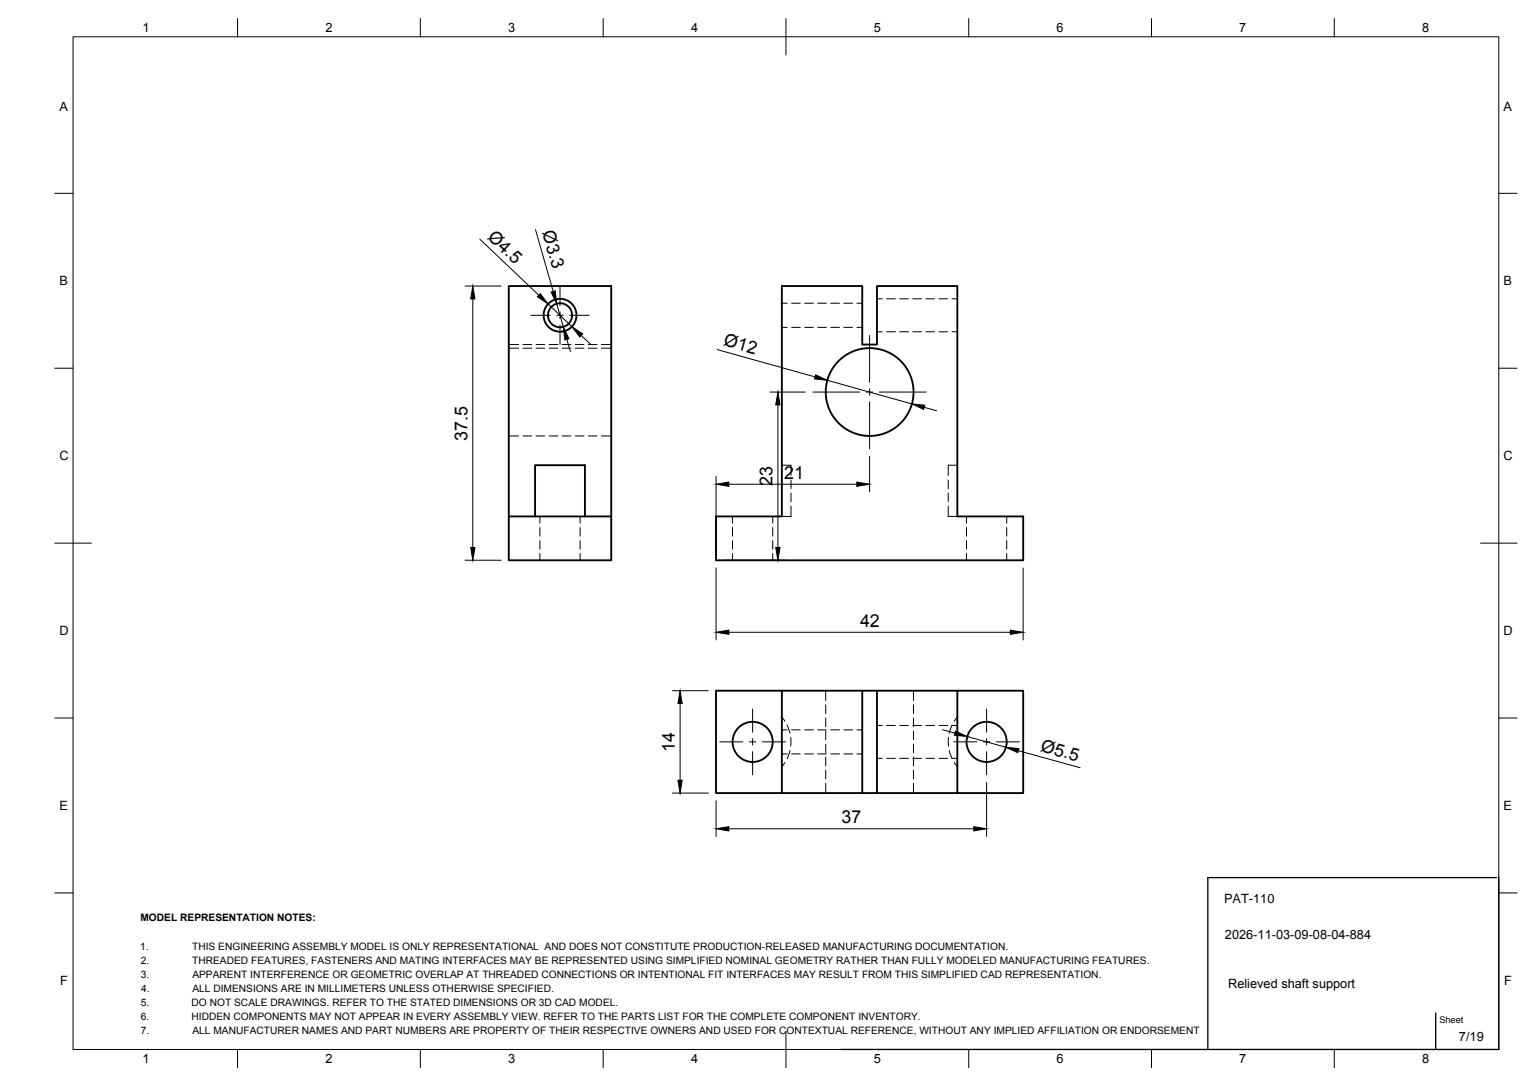
ISO-10303-21;
HEADER;
/* Generated by software containing ST-Developer
 * from STEP Tools, Inc. (www.steptools.com) 
 */

FILE_DESCRIPTION(
/* description */ ('Twin-shaft manual slide'),
/* implementation_level */ '2;1');

FILE_NAME(
/* name */ 'Relieved shaft support.step',
/* time_stamp */ '2026-10-27T18:38:08-07:00',
/* author */ (''),
/* organization */ (''),
/* preprocessor_version */ 'ST-DEVELOPER v20.2',
/* originating_system */ 'Autodesk Translation Framework v15.17.0.0',
/* authorisation */ '');

FILE_SCHEMA (('AUTOMOTIVE_DESIGN { 1 0 10303 214 3 1 1 }'));
ENDSEC;

DATA;
#10=MECHANICAL_DESIGN_GEOMETRIC_PRESENTATION_REPRESENTATION('',(#278),#6463);
#246=SHAPE_REPRESENTATION_RELATIONSHIP('SRR','None',#6564,#262);
#262=ADVANCED_BREP_SHAPE_REPRESENTATION('',(#294),#6447);
#278=STYLED_ITEM('',(#6740),#294);
#294=MANIFOLD_SOLID_BREP('Body1',#3640);
#328=FACE_BOUND('',#785,.T.);
#329=FACE_BOUND('',#787,.T.);
#330=FACE_BOUND('',#789,.T.);
#331=FACE_BOUND('',#796,.T.);
#332=FACE_BOUND('',#799,.T.);
#333=FACE_BOUND('',#800,.T.);
#334=FACE_BOUND('',#803,.T.);
#335=FACE_BOUND('',#806,.T.);
#336=FACE_BOUND('',#809,.T.);
#337=FACE_BOUND('',#812,.T.);
#409=PLANE('',#3891);
#410=PLANE('',#3898);
#411=PLANE('',#3899);
#412=PLANE('',#3901);
#413=PLANE('',#3903);
#414=PLANE('',#3917);
#415=PLANE('',#3918);
#416=PLANE('',#3919);
#417=PLANE('',#3920);
#418=PLANE('',#3921);
#419=PLANE('',#3922);
#420=PLANE('',#3923);
#421=PLANE('',#3924);
#422=PLANE('',#3925);
#423=PLANE('',#3926);
#424=PLANE('',#3927);
#549=FACE_OUTER_BOUND('',#780,.T.);
#550=FACE_OUTER_BOUND('',#781,.T.);
#551=FACE_OUTER_BOUND('',#782,.T.);
#552=FACE_OUTER_BOUND('',#783,.T.);
#553=FACE_OUTER_BOUND('',#784,.T.);
#554=FACE_OUTER_BOUND('',#786,.T.);
#555=FACE_OUTER_BOUND('',#788,.T.);
#556=FACE_OUTER_BOUND('',#790,.T.);
#557=FACE_OUTER_BOUND('',#791,.T.);
#558=FACE_OUTER_BOUND('',#792,.T.);
#559=FACE_OUTER_BOUND('',#793,.T.);
#560=FACE_OUTER_BOUND('',#794,.T.);
#561=FACE_OUTER_BOUND('',#795,.T.);
#562=FACE_OUTER_BOUND('',#797,.T.);
#563=FACE_OUTER_BOUND('',#798,.T.);
#564=FACE_OUTER_BOUND('',#801,.T.);
#565=FACE_OUTER_BOUND('',#802,.T.);
#566=FACE_OUTER_BOUND('',#804,.T.);
#567=FACE_OUTER_BOUND('',#805,.T.);
#568=FACE_OUTER_BOUND('',#807,.T.);
#569=FACE_OUTER_BOUND('',#808,.T.);
#570=FACE_OUTER_BOUND('',#810,.T.);
#571=FACE_OUTER_BOUND('',#811,.T.);
#780=EDGE_LOOP('',(#2598,#2599));
#781=EDGE_LOOP('',(#2600,#2601,#2602,#2603));
#782=EDGE_LOOP('',(#2604,#2605,#2606,#2607));
#783=EDGE_LOOP('',(#2608,#2609));
#784=EDGE_LOOP('',(#2610,#2611,#2612,#2613,#2614,#2615));
#785=EDGE_LOOP('',(#2616));
#786=EDGE_LOOP('',(#2617,#2618,#2619,#2620,#2621,#2622,#2623,#2624));
#787=EDGE_LOOP('',(#2625));
#788=EDGE_LOOP('',(#2626,#2627,#2628,#2629,#2630,#2631));
#789=EDGE_LOOP('',(#2632));
#790=EDGE_LOOP('',(#2633,#2634,#2635,#2636));
#791=EDGE_LOOP('',(#2637,#2638,#2639,#2640));
#792=EDGE_LOOP('',(#2641,#2642,#2643,#2644));
#793=EDGE_LOOP('',(#2645,#2646,#2647,#2648));
#794=EDGE_LOOP('',(#2649,#2650,#2651,#2652));
#795=EDGE_LOOP('',(#2653,#2654,#2655,#2656,#2657,#2658,#2659,#2660,#2661,
#2662,#2663,#2664));
#796=EDGE_LOOP('',(#2665));
#797=EDGE_LOOP('',(#2666,#2667,#2668,#2669));
#798=EDGE_LOOP('',(#2670,#2671,#2672,#2673));
#799=EDGE_LOOP('',(#2674));
#800=EDGE_LOOP('',(#2675));
#801=EDGE_LOOP('',(#2676,#2677,#2678,#2679));
#802=EDGE_LOOP('',(#2680,#2681,#2682,#2683,#2684,#2685,#2686,#2687));
#803=EDGE_LOOP('',(#2688));
#804=EDGE_LOOP('',(#2689,#2690,#2691,#2692));
#805=EDGE_LOOP('',(#2693,#2694,#2695,#2696));
#806=EDGE_LOOP('',(#2697));
#807=EDGE_LOOP('',(#2698,#2699,#2700,#2701));
#808=EDGE_LOOP('',(#2702,#2703,#2704,#2705));
#809=EDGE_LOOP('',(#2706));
#810=EDGE_LOOP('',(#2707,#2708,#2709,#2710));
#811=EDGE_LOOP('',(#2711,#2712,#2713,#2714,#2715,#2716,#2717,#2718,#2719,
#2720,#2721,#2722));
#812=EDGE_LOOP('',(#2723));
#1064=LINE('',#5539,#1350);
#1065=LINE('',#5543,#1351);
#1066=LINE('',#5546,#1352);
#1067=LINE('',#5550,#1353);
#1068=LINE('',#5554,#1354);
#1069=LINE('',#5557,#1355);
#1070=LINE('',#5560,#1356);
#1071=LINE('',#5562,#1357);
#1072=LINE('',#5564,#1358);
#1073=LINE('',#5566,#1359);
#1074=LINE('',#5567,#1360);
#1075=LINE('',#5572,#1361);
#1076=LINE('',#5574,#1362);
#1077=LINE('',#5575,#1363);
#1078=LINE('',#5581,#1364);
#1079=LINE('',#5583,#1365);
#1080=LINE('',#5584,#1366);
#1081=LINE('',#5586,#1367);
#1082=LINE('',#5587,#1368);
#1083=LINE('',#5594,#1369);
#1084=LINE('',#5598,#1370);
#1085=LINE('',#5603,#1371);
#1086=LINE('',#5607,#1372);
#1087=LINE('',#5612,#1373);
#1088=LINE('',#5616,#1374);
#1089=LINE('',#5618,#1375);
#1090=LINE('',#5619,#1376);
#1091=LINE('',#5621,#1377);
#1092=LINE('',#5623,#1378);
#1093=LINE('',#5625,#1379);
#1094=LINE('',#5627,#1380);
#1095=LINE('',#5629,#1381);
#1096=LINE('',#5630,#1382);
#1097=LINE('',#5633,#1383);
#1098=LINE('',#5634,#1384);
#1099=LINE('',#5637,#1385);
#1100=LINE('',#5638,#1386);
#1101=LINE('',#5640,#1387);
#1102=LINE('',#5643,#1388);
#1103=LINE('',#5644,#1389);
#1104=LINE('',#5647,#1390);
#1105=LINE('',#5648,#1391);
#1106=LINE('',#5651,#1392);
#1107=LINE('',#5652,#1393);
#1108=LINE('',#5655,#1394);
#1109=LINE('',#5656,#1395);
#1110=LINE('',#5659,#1396);
#1111=LINE('',#5660,#1397);
#1112=LINE('',#5662,#1398);
#1350=VECTOR('',#4408,1.);
#1351=VECTOR('',#4413,1.);
#1352=VECTOR('',#4416,1.);
#1353=VECTOR('',#4419,1.);
#1354=VECTOR('',#4422,1.);
#1355=VECTOR('',#4427,1.);
#1356=VECTOR('',#4430,1.);
#1357=VECTOR('',#4431,1.);
#1358=VECTOR('',#4432,1.);
#1359=VECTOR('',#4433,1.);
#1360=VECTOR('',#4434,1.);
#1361=VECTOR('',#4439,1.);
#1362=VECTOR('',#4440,1.);
#1363=VECTOR('',#4441,1.);
#1364=VECTOR('',#4446,1.);
#1365=VECTOR('',#4447,1.);
#1366=VECTOR('',#4448,1.);
#1367=VECTOR('',#4449,1.);
#1368=VECTOR('',#4450,1.);
#1369=VECTOR('',#4457,0.225);
#1370=VECTOR('',#4462,0.165);
#1371=VECTOR('',#4469,0.275);
#1372=VECTOR('',#4474,0.275);
#1373=VECTOR('',#4479,0.6);
#1374=VECTOR('',#4484,1.);
#1375=VECTOR('',#4485,1.);
#1376=VECTOR('',#4486,1.);
#1377=VECTOR('',#4487,1.);
#1378=VECTOR('',#4488,1.);
#1379=VECTOR('',#4489,1.);
#1380=VECTOR('',#4490,1.);
#1381=VECTOR('',#4491,1.);
#1382=VECTOR('',#4492,1.);
#1383=VECTOR('',#4495,1.);
#1384=VECTOR('',#4496,1.);
#1385=VECTOR('',#4499,1.);
#1386=VECTOR('',#4500,1.);
#1387=VECTOR('',#4503,1.);
#1388=VECTOR('',#4506,1.);
#1389=VECTOR('',#4507,1.);
#1390=VECTOR('',#4510,1.);
#1391=VECTOR('',#4511,1.);
#1392=VECTOR('',#4514,1.);
#1393=VECTOR('',#4515,1.);
#1394=VECTOR('',#4518,1.);
#1395=VECTOR('',#4519,1.);
#1396=VECTOR('',#4522,1.);
#1397=VECTOR('',#4523,1.);
#1398=VECTOR('',#4526,1.);
#1637=CIRCLE('',#3892,0.525);
#1638=CIRCLE('',#3894,0.525);
#1639=CIRCLE('',#3896,0.525);
#1640=CIRCLE('',#3897,0.525);
#1641=CIRCLE('',#3900,0.275);
#1642=CIRCLE('',#3902,0.165);
#1643=CIRCLE('',#3904,0.275);
#1644=CIRCLE('',#3906,0.225);
#1645=CIRCLE('',#3907,0.225);
#1646=CIRCLE('',#3909,0.165);
#1647=CIRCLE('',#3911,0.275);
#1648=CIRCLE('',#3913,0.275);
#1649=CIRCLE('',#3915,0.6);
#1650=CIRCLE('',#3916,0.6);
#1798=VERTEX_POINT('',#5537);
#1799=VERTEX_POINT('',#5538);
#1800=VERTEX_POINT('',#5542);
#1801=VERTEX_POINT('',#5544);
#1802=VERTEX_POINT('',#5548);
#1803=VERTEX_POINT('',#5549);
#1804=VERTEX_POINT('',#5551);
#1805=VERTEX_POINT('',#5553);
#1806=VERTEX_POINT('',#5559);
#1807=VERTEX_POINT('',#5561);
#1808=VERTEX_POINT('',#5563);
#1809=VERTEX_POINT('',#5565);
#1810=VERTEX_POINT('',#5568);
#1811=VERTEX_POINT('',#5571);
#1812=VERTEX_POINT('',#5573);
#1813=VERTEX_POINT('',#5576);
#1814=VERTEX_POINT('',#5579);
#1815=VERTEX_POINT('',#5580);
#1816=VERTEX_POINT('',#5582);
#1817=VERTEX_POINT('',#5585);
#1818=VERTEX_POINT('',#5588);
#1819=VERTEX_POINT('',#5591);
#1820=VERTEX_POINT('',#5593);
#1821=VERTEX_POINT('',#5597);
#1822=VERTEX_POINT('',#5601);
#1823=VERTEX_POINT('',#5605);
#1824=VERTEX_POINT('',#5609);
#1825=VERTEX_POINT('',#5611);
#1826=VERTEX_POINT('',#5615);
#1827=VERTEX_POINT('',#5617);
#1828=VERTEX_POINT('',#5620);
#1829=VERTEX_POINT('',#5622);
#1830=VERTEX_POINT('',#5624);
#1831=VERTEX_POINT('',#5626);
#1832=VERTEX_POINT('',#5628);
#1833=VERTEX_POINT('',#5632);
#1834=VERTEX_POINT('',#5636);
#1835=VERTEX_POINT('',#5642);
#1836=VERTEX_POINT('',#5646);
#1837=VERTEX_POINT('',#5650);
#1838=VERTEX_POINT('',#5654);
#1839=VERTEX_POINT('',#5658);
#2104=EDGE_CURVE('',#1798,#1799,#1064,.T.);
#2105=EDGE_CURVE('',#1799,#1798,#1637,.T.);
#2106=EDGE_CURVE('',#1800,#1798,#1065,.T.);
#2107=EDGE_CURVE('',#1801,#1800,#1638,.T.);
#2108=EDGE_CURVE('',#1799,#1801,#1066,.T.);
#2109=EDGE_CURVE('',#1802,#1803,#1067,.T.);
#2110=EDGE_CURVE('',#1802,#1804,#1639,.T.);
#2111=EDGE_CURVE('',#1805,#1804,#1068,.T.);
#2112=EDGE_CURVE('',#1803,#1805,#1640,.T.);
#2113=EDGE_CURVE('',#1804,#1802,#1069,.T.);
#2114=EDGE_CURVE('',#1800,#1806,#1070,.T.);
#2115=EDGE_CURVE('',#1807,#1806,#1071,.T.);
#2116=EDGE_CURVE('',#1807,#1808,#1072,.T.);
#2117=EDGE_CURVE('',#1809,#1808,#1073,.T.);
#2118=EDGE_CURVE('',#1809,#1801,#1074,.T.);
#2119=EDGE_CURVE('',#1810,#1810,#1641,.T.);
#2120=EDGE_CURVE('',#1811,#1809,#1075,.T.);
#2121=EDGE_CURVE('',#1811,#1812,#1076,.T.);
#2122=EDGE_CURVE('',#1806,#1812,#1077,.T.);
#2123=EDGE_CURVE('',#1813,#1813,#1642,.T.);
#2124=EDGE_CURVE('',#1814,#1815,#1078,.T.);
#2125=EDGE_CURVE('',#1816,#1815,#1079,.T.);
#2126=EDGE_CURVE('',#1803,#1816,#1080,.T.);
#2127=EDGE_CURVE('',#1817,#1805,#1081,.T.);
#2128=EDGE_CURVE('',#1814,#1817,#1082,.T.);
#2129=EDGE_CURVE('',#1818,#1818,#1643,.T.);
#2130=EDGE_CURVE('',#1819,#1819,#1644,.T.);
#2131=EDGE_CURVE('',#1819,#1820,#1083,.T.);
#2132=EDGE_CURVE('',#1820,#1820,#1645,.T.);
#2133=EDGE_CURVE('',#1813,#1821,#1084,.T.);
#2134=EDGE_CURVE('',#1821,#1821,#1646,.T.);
#2135=EDGE_CURVE('',#1822,#1822,#1647,.T.);
#2136=EDGE_CURVE('',#1822,#1810,#1085,.T.);
#2137=EDGE_CURVE('',#1823,#1823,#1648,.T.);
#2138=EDGE_CURVE('',#1823,#1818,#1086,.T.);
#2139=EDGE_CURVE('',#1824,#1824,#1649,.T.);
#2140=EDGE_CURVE('',#1824,#1825,#1087,.T.);
#2141=EDGE_CURVE('',#1825,#1825,#1650,.T.);
#2142=EDGE_CURVE('',#1808,#1826,#1088,.T.);
#2143=EDGE_CURVE('',#1826,#1827,#1089,.T.);
#2144=EDGE_CURVE('',#1827,#1814,#1090,.T.);
#2145=EDGE_CURVE('',#1817,#1828,#1091,.T.);
#2146=EDGE_CURVE('',#1828,#1829,#1092,.T.);
#2147=EDGE_CURVE('',#1829,#1830,#1093,.T.);
#2148=EDGE_CURVE('',#1830,#1831,#1094,.T.);
#2149=EDGE_CURVE('',#1831,#1832,#1095,.T.);
#2150=EDGE_CURVE('',#1832,#1811,#1096,.T.);
#2151=EDGE_CURVE('',#1833,#1807,#1097,.T.);
#2152=EDGE_CURVE('',#1826,#1833,#1098,.T.);
#2153=EDGE_CURVE('',#1834,#1833,#1099,.T.);
#2154=EDGE_CURVE('',#1827,#1834,#1100,.T.);
#2155=EDGE_CURVE('',#1815,#1834,#1101,.T.);
#2156=EDGE_CURVE('',#1835,#1816,#1102,.T.);
#2157=EDGE_CURVE('',#1828,#1835,#1103,.T.);
#2158=EDGE_CURVE('',#1836,#1835,#1104,.T.);
#2159=EDGE_CURVE('',#1829,#1836,#1105,.T.);
#2160=EDGE_CURVE('',#1837,#1836,#1106,.T.);
#2161=EDGE_CURVE('',#1830,#1837,#1107,.T.);
#2162=EDGE_CURVE('',#1838,#1837,#1108,.T.);
#2163=EDGE_CURVE('',#1831,#1838,#1109,.T.);
#2164=EDGE_CURVE('',#1839,#1838,#1110,.T.);
#2165=EDGE_CURVE('',#1832,#1839,#1111,.T.);
#2166=EDGE_CURVE('',#1812,#1839,#1112,.T.);
#2598=ORIENTED_EDGE('',*,*,#2104,.F.);
#2599=ORIENTED_EDGE('',*,*,#2105,.F.);
#2600=ORIENTED_EDGE('',*,*,#2106,.F.);
#2601=ORIENTED_EDGE('',*,*,#2107,.F.);
#2602=ORIENTED_EDGE('',*,*,#2108,.F.);
#2603=ORIENTED_EDGE('',*,*,#2105,.T.);
#2604=ORIENTED_EDGE('',*,*,#2109,.F.);
#2605=ORIENTED_EDGE('',*,*,#2110,.T.);
#2606=ORIENTED_EDGE('',*,*,#2111,.F.);
#2607=ORIENTED_EDGE('',*,*,#2112,.F.);
#2608=ORIENTED_EDGE('',*,*,#2113,.F.);
#2609=ORIENTED_EDGE('',*,*,#2110,.F.);
#2610=ORIENTED_EDGE('',*,*,#2114,.T.);
#2611=ORIENTED_EDGE('',*,*,#2115,.F.);
#2612=ORIENTED_EDGE('',*,*,#2116,.T.);
#2613=ORIENTED_EDGE('',*,*,#2117,.F.);
#2614=ORIENTED_EDGE('',*,*,#2118,.T.);
#2615=ORIENTED_EDGE('',*,*,#2107,.T.);
#2616=ORIENTED_EDGE('',*,*,#2119,.T.);
#2617=ORIENTED_EDGE('',*,*,#2106,.T.);
#2618=ORIENTED_EDGE('',*,*,#2104,.T.);
#2619=ORIENTED_EDGE('',*,*,#2108,.T.);
#2620=ORIENTED_EDGE('',*,*,#2118,.F.);
#2621=ORIENTED_EDGE('',*,*,#2120,.F.);
#2622=ORIENTED_EDGE('',*,*,#2121,.T.);
#2623=ORIENTED_EDGE('',*,*,#2122,.F.);
#2624=ORIENTED_EDGE('',*,*,#2114,.F.);
#2625=ORIENTED_EDGE('',*,*,#2123,.T.);
#2626=ORIENTED_EDGE('',*,*,#2124,.T.);
#2627=ORIENTED_EDGE('',*,*,#2125,.F.);
#2628=ORIENTED_EDGE('',*,*,#2126,.F.);
#2629=ORIENTED_EDGE('',*,*,#2112,.T.);
#2630=ORIENTED_EDGE('',*,*,#2127,.F.);
#2631=ORIENTED_EDGE('',*,*,#2128,.F.);
#2632=ORIENTED_EDGE('',*,*,#2129,.T.);
#2633=ORIENTED_EDGE('',*,*,#2130,.F.);
#2634=ORIENTED_EDGE('',*,*,#2131,.T.);
#2635=ORIENTED_EDGE('',*,*,#2132,.F.);
#2636=ORIENTED_EDGE('',*,*,#2131,.F.);
#2637=ORIENTED_EDGE('',*,*,#2123,.F.);
#2638=ORIENTED_EDGE('',*,*,#2133,.T.);
#2639=ORIENTED_EDGE('',*,*,#2134,.F.);
#2640=ORIENTED_EDGE('',*,*,#2133,.F.);
#2641=ORIENTED_EDGE('',*,*,#2135,.F.);
#2642=ORIENTED_EDGE('',*,*,#2136,.T.);
#2643=ORIENTED_EDGE('',*,*,#2119,.F.);
#2644=ORIENTED_EDGE('',*,*,#2136,.F.);
#2645=ORIENTED_EDGE('',*,*,#2137,.F.);
#2646=ORIENTED_EDGE('',*,*,#2138,.T.);
#2647=ORIENTED_EDGE('',*,*,#2129,.F.);
#2648=ORIENTED_EDGE('',*,*,#2138,.F.);
#2649=ORIENTED_EDGE('',*,*,#2139,.F.);
#2650=ORIENTED_EDGE('',*,*,#2140,.T.);
#2651=ORIENTED_EDGE('',*,*,#2141,.F.);
#2652=ORIENTED_EDGE('',*,*,#2140,.F.);
#2653=ORIENTED_EDGE('',*,*,#2117,.T.);
#2654=ORIENTED_EDGE('',*,*,#2142,.T.);
#2655=ORIENTED_EDGE('',*,*,#2143,.T.);
#2656=ORIENTED_EDGE('',*,*,#2144,.T.);
#2657=ORIENTED_EDGE('',*,*,#2128,.T.);
#2658=ORIENTED_EDGE('',*,*,#2145,.T.);
#2659=ORIENTED_EDGE('',*,*,#2146,.T.);
#2660=ORIENTED_EDGE('',*,*,#2147,.T.);
#2661=ORIENTED_EDGE('',*,*,#2148,.T.);
#2662=ORIENTED_EDGE('',*,*,#2149,.T.);
#2663=ORIENTED_EDGE('',*,*,#2150,.T.);
#2664=ORIENTED_EDGE('',*,*,#2120,.T.);
#2665=ORIENTED_EDGE('',*,*,#2139,.T.);
#2666=ORIENTED_EDGE('',*,*,#2116,.F.);
#2667=ORIENTED_EDGE('',*,*,#2151,.F.);
#2668=ORIENTED_EDGE('',*,*,#2152,.F.);
#2669=ORIENTED_EDGE('',*,*,#2142,.F.);
#2670=ORIENTED_EDGE('',*,*,#2152,.T.);
#2671=ORIENTED_EDGE('',*,*,#2153,.F.);
#2672=ORIENTED_EDGE('',*,*,#2154,.F.);
#2673=ORIENTED_EDGE('',*,*,#2143,.F.);
#2674=ORIENTED_EDGE('',*,*,#2135,.T.);
#2675=ORIENTED_EDGE('',*,*,#2137,.T.);
#2676=ORIENTED_EDGE('',*,*,#2154,.T.);
#2677=ORIENTED_EDGE('',*,*,#2155,.F.);
#2678=ORIENTED_EDGE('',*,*,#2124,.F.);
#2679=ORIENTED_EDGE('',*,*,#2144,.F.);
#2680=ORIENTED_EDGE('',*,*,#2109,.T.);
#2681=ORIENTED_EDGE('',*,*,#2126,.T.);
#2682=ORIENTED_EDGE('',*,*,#2156,.F.);
#2683=ORIENTED_EDGE('',*,*,#2157,.F.);
#2684=ORIENTED_EDGE('',*,*,#2145,.F.);
#2685=ORIENTED_EDGE('',*,*,#2127,.T.);
#2686=ORIENTED_EDGE('',*,*,#2111,.T.);
#2687=ORIENTED_EDGE('',*,*,#2113,.T.);
#2688=ORIENTED_EDGE('',*,*,#2132,.T.);
#2689=ORIENTED_EDGE('',*,*,#2157,.T.);
#2690=ORIENTED_EDGE('',*,*,#2158,.F.);
#2691=ORIENTED_EDGE('',*,*,#2159,.F.);
#2692=ORIENTED_EDGE('',*,*,#2146,.F.);
#2693=ORIENTED_EDGE('',*,*,#2159,.T.);
#2694=ORIENTED_EDGE('',*,*,#2160,.F.);
#2695=ORIENTED_EDGE('',*,*,#2161,.F.);
#2696=ORIENTED_EDGE('',*,*,#2147,.F.);
#2697=ORIENTED_EDGE('',*,*,#2130,.T.);
#2698=ORIENTED_EDGE('',*,*,#2161,.T.);
#2699=ORIENTED_EDGE('',*,*,#2162,.F.);
#2700=ORIENTED_EDGE('',*,*,#2163,.F.);
#2701=ORIENTED_EDGE('',*,*,#2148,.F.);
#2702=ORIENTED_EDGE('',*,*,#2163,.T.);
#2703=ORIENTED_EDGE('',*,*,#2164,.F.);
#2704=ORIENTED_EDGE('',*,*,#2165,.F.);
#2705=ORIENTED_EDGE('',*,*,#2149,.F.);
#2706=ORIENTED_EDGE('',*,*,#2134,.T.);
#2707=ORIENTED_EDGE('',*,*,#2165,.T.);
#2708=ORIENTED_EDGE('',*,*,#2166,.F.);
#2709=ORIENTED_EDGE('',*,*,#2121,.F.);
#2710=ORIENTED_EDGE('',*,*,#2150,.F.);
#2711=ORIENTED_EDGE('',*,*,#2115,.T.);
#2712=ORIENTED_EDGE('',*,*,#2122,.T.);
#2713=ORIENTED_EDGE('',*,*,#2166,.T.);
#2714=ORIENTED_EDGE('',*,*,#2164,.T.);
#2715=ORIENTED_EDGE('',*,*,#2162,.T.);
#2716=ORIENTED_EDGE('',*,*,#2160,.T.);
#2717=ORIENTED_EDGE('',*,*,#2158,.T.);
#2718=ORIENTED_EDGE('',*,*,#2156,.T.);
#2719=ORIENTED_EDGE('',*,*,#2125,.T.);
#2720=ORIENTED_EDGE('',*,*,#2155,.T.);
#2721=ORIENTED_EDGE('',*,*,#2153,.T.);
#2722=ORIENTED_EDGE('',*,*,#2151,.T.);
#2723=ORIENTED_EDGE('',*,*,#2141,.T.);
#3379=CYLINDRICAL_SURFACE('',#3893,0.525);
#3380=CYLINDRICAL_SURFACE('',#3895,0.525);
#3381=CYLINDRICAL_SURFACE('',#3905,0.225);
#3382=CYLINDRICAL_SURFACE('',#3908,0.165);
#3383=CYLINDRICAL_SURFACE('',#3910,0.275);
#3384=CYLINDRICAL_SURFACE('',#3912,0.275);
#3385=CYLINDRICAL_SURFACE('',#3914,0.6);
#3454=ADVANCED_FACE('',(#549),#409,.F.);
#3455=ADVANCED_FACE('',(#550),#3379,.F.);
#3456=ADVANCED_FACE('',(#551),#3380,.F.);
#3457=ADVANCED_FACE('',(#552),#410,.F.);
#3458=ADVANCED_FACE('',(#553,#328),#411,.T.);
#3459=ADVANCED_FACE('',(#554,#329),#412,.T.);
#3460=ADVANCED_FACE('',(#555,#330),#413,.T.);
#3461=ADVANCED_FACE('',(#556),#3381,.F.);
#3462=ADVANCED_FACE('',(#557),#3382,.F.);
#3463=ADVANCED_FACE('',(#558),#3383,.F.);
#3464=ADVANCED_FACE('',(#559),#3384,.F.);
#3465=ADVANCED_FACE('',(#560),#3385,.F.);
#3466=ADVANCED_FACE('',(#561,#331),#414,.T.);
#3467=ADVANCED_FACE('',(#562),#415,.T.);
#3468=ADVANCED_FACE('',(#563,#332,#333),#416,.T.);
#3469=ADVANCED_FACE('',(#564),#417,.T.);
#3470=ADVANCED_FACE('',(#565,#334),#418,.T.);
#3471=ADVANCED_FACE('',(#566),#419,.T.);
#3472=ADVANCED_FACE('',(#567,#335),#420,.T.);
#3473=ADVANCED_FACE('',(#568),#421,.T.);
#3474=ADVANCED_FACE('',(#569,#336),#422,.T.);
#3475=ADVANCED_FACE('',(#570),#423,.T.);
#3476=ADVANCED_FACE('',(#571,#337),#424,.T.);
#3640=CLOSED_SHELL('',(#3454,#3455,#3456,#3457,#3458,#3459,#3460,#3461,
#3462,#3463,#3464,#3465,#3466,#3467,#3468,#3469,#3470,#3471,#3472,#3473,
#3474,#3475,#3476));
#3890=AXIS2_PLACEMENT_3D('',#5535,#4404,#4405);
#3891=AXIS2_PLACEMENT_3D('',#5536,#4406,#4407);
#3892=AXIS2_PLACEMENT_3D('',#5540,#4409,#4410);
#3893=AXIS2_PLACEMENT_3D('',#5541,#4411,#4412);
#3894=AXIS2_PLACEMENT_3D('',#5545,#4414,#4415);
#3895=AXIS2_PLACEMENT_3D('',#5547,#4417,#4418);
#3896=AXIS2_PLACEMENT_3D('',#5552,#4420,#4421);
#3897=AXIS2_PLACEMENT_3D('',#5555,#4423,#4424);
#3898=AXIS2_PLACEMENT_3D('',#5556,#4425,#4426);
#3899=AXIS2_PLACEMENT_3D('',#5558,#4428,#4429);
#3900=AXIS2_PLACEMENT_3D('',#5569,#4435,#4436);
#3901=AXIS2_PLACEMENT_3D('',#5570,#4437,#4438);
#3902=AXIS2_PLACEMENT_3D('',#5577,#4442,#4443);
#3903=AXIS2_PLACEMENT_3D('',#5578,#4444,#4445);
#3904=AXIS2_PLACEMENT_3D('',#5589,#4451,#4452);
#3905=AXIS2_PLACEMENT_3D('',#5590,#4453,#4454);
#3906=AXIS2_PLACEMENT_3D('',#5592,#4455,#4456);
#3907=AXIS2_PLACEMENT_3D('',#5595,#4458,#4459);
#3908=AXIS2_PLACEMENT_3D('',#5596,#4460,#4461);
#3909=AXIS2_PLACEMENT_3D('',#5599,#4463,#4464);
#3910=AXIS2_PLACEMENT_3D('',#5600,#4465,#4466);
#3911=AXIS2_PLACEMENT_3D('',#5602,#4467,#4468);
#3912=AXIS2_PLACEMENT_3D('',#5604,#4470,#4471);
#3913=AXIS2_PLACEMENT_3D('',#5606,#4472,#4473);
#3914=AXIS2_PLACEMENT_3D('',#5608,#4475,#4476);
#3915=AXIS2_PLACEMENT_3D('',#5610,#4477,#4478);
#3916=AXIS2_PLACEMENT_3D('',#5613,#4480,#4481);
#3917=AXIS2_PLACEMENT_3D('',#5614,#4482,#4483);
#3918=AXIS2_PLACEMENT_3D('',#5631,#4493,#4494);
#3919=AXIS2_PLACEMENT_3D('',#5635,#4497,#4498);
#3920=AXIS2_PLACEMENT_3D('',#5639,#4501,#4502);
#3921=AXIS2_PLACEMENT_3D('',#5641,#4504,#4505);
#3922=AXIS2_PLACEMENT_3D('',#5645,#4508,#4509);
#3923=AXIS2_PLACEMENT_3D('',#5649,#4512,#4513);
#3924=AXIS2_PLACEMENT_3D('',#5653,#4516,#4517);
#3925=AXIS2_PLACEMENT_3D('',#5657,#4520,#4521);
#3926=AXIS2_PLACEMENT_3D('',#5661,#4524,#4525);
#3927=AXIS2_PLACEMENT_3D('',#5663,#4527,#4528);
#4404=DIRECTION('axis',(0.,0.,1.));
#4405=DIRECTION('refdir',(1.,0.,0.));
#4406=DIRECTION('center_axis',(0.,0.,1.));
#4407=DIRECTION('ref_axis',(1.,0.,0.));
#4408=DIRECTION('',(0.,-1.,0.));
#4409=DIRECTION('center_axis',(0.,0.,1.));
#4410=DIRECTION('ref_axis',(1.,0.,0.));
#4411=DIRECTION('center_axis',(0.,0.,1.));
#4412=DIRECTION('ref_axis',(1.,0.,0.));
#4413=DIRECTION('',(0.,0.,1.));
#4414=DIRECTION('center_axis',(0.,0.,1.));
#4415=DIRECTION('ref_axis',(1.,0.,0.));
#4416=DIRECTION('',(0.,0.,-1.));
#4417=DIRECTION('center_axis',(0.,0.,1.));
#4418=DIRECTION('ref_axis',(-1.,1.22464679914735E-16,0.));
#4419=DIRECTION('',(0.,0.,-1.));
#4420=DIRECTION('center_axis',(0.,0.,1.));
#4421=DIRECTION('ref_axis',(1.,0.,0.));
#4422=DIRECTION('',(0.,0.,1.));
#4423=DIRECTION('center_axis',(0.,0.,1.));
#4424=DIRECTION('ref_axis',(1.,0.,0.));
#4425=DIRECTION('center_axis',(0.,0.,1.));
#4426=DIRECTION('ref_axis',(1.,0.,0.));
#4427=DIRECTION('',(0.,1.,0.));
#4428=DIRECTION('center_axis',(0.,0.,1.));
#4429=DIRECTION('ref_axis',(1.,0.,0.));
#4430=DIRECTION('',(0.,1.,0.));
#4431=DIRECTION('',(1.,0.,0.));
#4432=DIRECTION('',(0.,-1.,0.));
#4433=DIRECTION('',(-1.,0.,0.));
#4434=DIRECTION('',(0.,1.,0.));
#4435=DIRECTION('center_axis',(0.,0.,-1.));
#4436=DIRECTION('ref_axis',(1.,0.,0.));
#4437=DIRECTION('center_axis',(-1.,0.,0.));
#4438=DIRECTION('ref_axis',(0.,0.,1.));
#4439=DIRECTION('',(0.,0.,-1.));
#4440=DIRECTION('',(0.,1.,0.));
#4441=DIRECTION('',(0.,0.,1.));
#4442=DIRECTION('center_axis',(1.,0.,0.));
#4443=DIRECTION('ref_axis',(0.,0.,-1.));
#4444=DIRECTION('center_axis',(0.,0.,1.));
#4445=DIRECTION('ref_axis',(1.,0.,0.));
#4446=DIRECTION('',(0.,1.,0.));
#4447=DIRECTION('',(1.,0.,0.));
#4448=DIRECTION('',(0.,1.,0.));
#4449=DIRECTION('',(0.,1.,0.));
#4450=DIRECTION('',(-1.,0.,0.));
#4451=DIRECTION('center_axis',(0.,0.,-1.));
#4452=DIRECTION('ref_axis',(1.,0.,0.));
#4453=DIRECTION('center_axis',(1.,0.,0.));
#4454=DIRECTION('ref_axis',(0.,0.,-1.));
#4455=DIRECTION('center_axis',(1.,0.,0.));
#4456=DIRECTION('ref_axis',(0.,0.,-1.));
#4457=DIRECTION('',(1.,0.,0.));
#4458=DIRECTION('center_axis',(-1.,0.,0.));
#4459=DIRECTION('ref_axis',(0.,0.,-1.));
#4460=DIRECTION('center_axis',(1.,0.,0.));
#4461=DIRECTION('ref_axis',(0.,0.,-1.));
#4462=DIRECTION('',(1.,0.,0.));
#4463=DIRECTION('center_axis',(-1.,0.,0.));
#4464=DIRECTION('ref_axis',(0.,0.,-1.));
#4465=DIRECTION('center_axis',(0.,0.,1.));
#4466=DIRECTION('ref_axis',(1.,0.,0.));
#4467=DIRECTION('center_axis',(0.,0.,1.));
#4468=DIRECTION('ref_axis',(1.,0.,0.));
#4469=DIRECTION('',(0.,0.,1.));
#4470=DIRECTION('center_axis',(0.,0.,1.));
#4471=DIRECTION('ref_axis',(1.,0.,0.));
#4472=DIRECTION('center_axis',(0.,0.,1.));
#4473=DIRECTION('ref_axis',(1.,0.,0.));
#4474=DIRECTION('',(0.,0.,1.));
#4475=DIRECTION('center_axis',(0.,1.,0.));
#4476=DIRECTION('ref_axis',(1.,0.,0.));
#4477=DIRECTION('center_axis',(0.,1.,0.));
#4478=DIRECTION('ref_axis',(1.,0.,0.));
#4479=DIRECTION('',(0.,1.,0.));
#4480=DIRECTION('center_axis',(0.,-1.,0.));
#4481=DIRECTION('ref_axis',(1.,0.,0.));
#4482=DIRECTION('center_axis',(0.,-1.,0.));
#4483=DIRECTION('ref_axis',(0.,0.,-1.));
#4484=DIRECTION('',(0.,0.,-1.));
#4485=DIRECTION('',(1.,0.,0.));
#4486=DIRECTION('',(0.,0.,1.));
#4487=DIRECTION('',(0.,0.,1.));
#4488=DIRECTION('',(-1.,0.,0.));
#4489=DIRECTION('',(0.,0.,-1.));
#4490=DIRECTION('',(-1.,0.,0.));
#4491=DIRECTION('',(0.,0.,1.));
#4492=DIRECTION('',(-1.,0.,0.));
#4493=DIRECTION('center_axis',(-1.,0.,0.));
#4494=DIRECTION('ref_axis',(0.,0.,1.));
#4495=DIRECTION('',(0.,0.,1.));
#4496=DIRECTION('',(0.,1.,0.));
#4497=DIRECTION('center_axis',(0.,0.,-1.));
#4498=DIRECTION('ref_axis',(-1.,0.,0.));
#4499=DIRECTION('',(-1.,0.,0.));
#4500=DIRECTION('',(0.,1.,0.));
#4501=DIRECTION('center_axis',(1.,0.,0.));
#4502=DIRECTION('ref_axis',(0.,0.,-1.));
#4503=DIRECTION('',(0.,0.,-1.));
#4504=DIRECTION('center_axis',(1.,0.,0.));
#4505=DIRECTION('ref_axis',(0.,0.,-1.));
#4506=DIRECTION('',(0.,0.,-1.));
#4507=DIRECTION('',(0.,1.,0.));
#4508=DIRECTION('center_axis',(0.,0.,1.));
#4509=DIRECTION('ref_axis',(1.,0.,0.));
#4510=DIRECTION('',(1.,0.,0.));
#4511=DIRECTION('',(0.,1.,0.));
#4512=DIRECTION('center_axis',(-1.,0.,0.));
#4513=DIRECTION('ref_axis',(0.,0.,1.));
#4514=DIRECTION('',(0.,0.,1.));
#4515=DIRECTION('',(0.,1.,0.));
#4516=DIRECTION('center_axis',(0.,0.,1.));
#4517=DIRECTION('ref_axis',(1.,0.,0.));
#4518=DIRECTION('',(1.,0.,0.));
#4519=DIRECTION('',(0.,1.,0.));
#4520=DIRECTION('center_axis',(1.,0.,0.));
#4521=DIRECTION('ref_axis',(0.,0.,-1.));
#4522=DIRECTION('',(0.,0.,-1.));
#4523=DIRECTION('',(0.,1.,0.));
#4524=DIRECTION('center_axis',(0.,0.,1.));
#4525=DIRECTION('ref_axis',(1.,0.,0.));
#4526=DIRECTION('',(1.,0.,0.));
#4527=DIRECTION('center_axis',(0.,1.,0.));
#4528=DIRECTION('ref_axis',(0.,0.,1.));
#5535=CARTESIAN_POINT('',(0.,0.,0.));
#5536=CARTESIAN_POINT('Origin',(-1.6,0.,1.3));
#5537=CARTESIAN_POINT('',(-1.2,0.340036762718386,1.3));
#5538=CARTESIAN_POINT('',(-1.2,-0.340036762718386,1.3));
#5539=CARTESIAN_POINT('',(-1.2,0.,1.3));
#5540=CARTESIAN_POINT('Origin',(-1.6,0.,1.3));
#5541=CARTESIAN_POINT('Origin',(-1.6,0.,0.6));
#5542=CARTESIAN_POINT('',(-1.2,0.340036762718386,0.6));
#5543=CARTESIAN_POINT('',(-1.2,0.340036762718386,0.6));
#5544=CARTESIAN_POINT('',(-1.2,-0.340036762718386,0.6));
#5545=CARTESIAN_POINT('Origin',(-1.6,0.,0.6));
#5546=CARTESIAN_POINT('',(-1.2,-0.340036762718386,0.6));
#5547=CARTESIAN_POINT('Origin',(1.6,0.,0.6));
#5548=CARTESIAN_POINT('',(1.2,0.340036762718386,1.3));
#5549=CARTESIAN_POINT('',(1.2,0.340036762718386,0.6));
#5550=CARTESIAN_POINT('',(1.2,0.340036762718386,0.6));
#5551=CARTESIAN_POINT('',(1.2,-0.340036762718386,1.3));
#5552=CARTESIAN_POINT('Origin',(1.6,0.,1.3));
#5553=CARTESIAN_POINT('',(1.2,-0.340036762718386,0.6));
#5554=CARTESIAN_POINT('',(1.2,-0.340036762718386,0.6));
#5555=CARTESIAN_POINT('Origin',(1.6,0.,0.6));
#5556=CARTESIAN_POINT('Origin',(1.6,0.,1.3));
#5557=CARTESIAN_POINT('',(1.2,0.,1.3));
#5558=CARTESIAN_POINT('Origin',(-2.1,0.,0.6));
#5559=CARTESIAN_POINT('',(-1.2,0.7,0.6));
#5560=CARTESIAN_POINT('',(-1.2,0.,0.6));
#5561=CARTESIAN_POINT('',(-2.1,0.7,0.6));
#5562=CARTESIAN_POINT('',(-1.2,0.7,0.6));
#5563=CARTESIAN_POINT('',(-2.1,-0.7,0.6));
#5564=CARTESIAN_POINT('',(-2.1,0.,0.6));
#5565=CARTESIAN_POINT('',(-1.2,-0.7,0.6));
#5566=CARTESIAN_POINT('',(-1.2,-0.7,0.6));
#5567=CARTESIAN_POINT('',(-1.2,0.,0.6));
#5568=CARTESIAN_POINT('',(-1.875,3.36777869765522E-17,0.6));
#5569=CARTESIAN_POINT('Origin',(-1.6,0.,0.6));
#5570=CARTESIAN_POINT('Origin',(-1.2,0.,0.6));
#5571=CARTESIAN_POINT('',(-1.2,-0.7,3.75));
#5572=CARTESIAN_POINT('',(-1.2,-0.7,3.75));
#5573=CARTESIAN_POINT('',(-1.2,0.7,3.75));
#5574=CARTESIAN_POINT('',(-1.2,0.,3.75));
#5575=CARTESIAN_POINT('',(-1.2,0.7,3.75));
#5576=CARTESIAN_POINT('',(-1.2,-2.02066721859313E-17,3.515));
#5577=CARTESIAN_POINT('Origin',(-1.2,0.,3.35));
#5578=CARTESIAN_POINT('Origin',(1.2,0.,0.6));
#5579=CARTESIAN_POINT('',(2.1,-0.7,0.6));
#5580=CARTESIAN_POINT('',(2.1,0.7,0.6));
#5581=CARTESIAN_POINT('',(2.1,0.,0.6));
#5582=CARTESIAN_POINT('',(1.2,0.7,0.6));
#5583=CARTESIAN_POINT('',(2.1,0.7,0.6));
#5584=CARTESIAN_POINT('',(1.2,0.,0.6));
#5585=CARTESIAN_POINT('',(1.2,-0.7,0.6));
#5586=CARTESIAN_POINT('',(1.2,0.,0.6));
#5587=CARTESIAN_POINT('',(2.1,-0.7,0.6));
#5588=CARTESIAN_POINT('',(1.325,3.36777869765522E-17,0.6));
#5589=CARTESIAN_POINT('Origin',(1.6,0.,0.6));
#5590=CARTESIAN_POINT('Origin',(0.1,0.,3.35));
#5591=CARTESIAN_POINT('',(0.1,-2.75545529808155E-17,3.575));
#5592=CARTESIAN_POINT('Origin',(0.1,0.,3.35));
#5593=CARTESIAN_POINT('',(1.2,2.75545529808155E-17,3.575));
#5594=CARTESIAN_POINT('',(0.1,-2.75545529808155E-17,3.575));
#5595=CARTESIAN_POINT('Origin',(1.2,0.,3.35));
#5596=CARTESIAN_POINT('Origin',(0.,0.,3.35));
#5597=CARTESIAN_POINT('',(-0.1,2.02066721859313E-17,3.515));
#5598=CARTESIAN_POINT('',(0.,-2.02066721859313E-17,3.515));
#5599=CARTESIAN_POINT('Origin',(-0.1,0.,3.35));
#5600=CARTESIAN_POINT('Origin',(-1.6,0.,-0.05));
#5601=CARTESIAN_POINT('',(-1.875,-3.36777869765522E-17,0.));
#5602=CARTESIAN_POINT('Origin',(-1.6,0.,0.));
#5603=CARTESIAN_POINT('',(-1.875,-3.36777869765522E-17,-0.05));
#5604=CARTESIAN_POINT('Origin',(1.6,0.,-0.05));
#5605=CARTESIAN_POINT('',(1.325,-3.36777869765522E-17,0.));
#5606=CARTESIAN_POINT('Origin',(1.6,0.,0.));
#5607=CARTESIAN_POINT('',(1.325,-3.36777869765522E-17,-0.05));
#5608=CARTESIAN_POINT('Origin',(0.,0.,2.3));
#5609=CARTESIAN_POINT('',(-0.6,-0.7,2.3));
#5610=CARTESIAN_POINT('Origin',(0.,-0.7,2.3));
#5611=CARTESIAN_POINT('',(-0.6,0.7,2.3));
#5612=CARTESIAN_POINT('',(-0.6,0.,2.3));
#5613=CARTESIAN_POINT('Origin',(0.,0.7,2.3));
#5614=CARTESIAN_POINT('Origin',(0.,-0.7,1.875));
#5615=CARTESIAN_POINT('',(-2.1,-0.7,0.));
#5616=CARTESIAN_POINT('',(-2.1,-0.7,0.6));
#5617=CARTESIAN_POINT('',(2.1,-0.7,0.));
#5618=CARTESIAN_POINT('',(-2.1,-0.7,0.));
#5619=CARTESIAN_POINT('',(2.1,-0.7,0.));
#5620=CARTESIAN_POINT('',(1.2,-0.7,3.75));
#5621=CARTESIAN_POINT('',(1.2,-0.7,0.6));
#5622=CARTESIAN_POINT('',(0.1,-0.7,3.75));
#5623=CARTESIAN_POINT('',(1.2,-0.7,3.75));
#5624=CARTESIAN_POINT('',(0.1,-0.7,2.95));
#5625=CARTESIAN_POINT('',(0.1,-0.7,3.75));
#5626=CARTESIAN_POINT('',(-0.1,-0.7,2.95));
#5627=CARTESIAN_POINT('',(0.1,-0.7,2.95));
#5628=CARTESIAN_POINT('',(-0.1,-0.7,3.75));
#5629=CARTESIAN_POINT('',(-0.1,-0.7,2.95));
#5630=CARTESIAN_POINT('',(-0.1,-0.7,3.75));
#5631=CARTESIAN_POINT('Origin',(-2.1,0.,0.));
#5632=CARTESIAN_POINT('',(-2.1,0.7,0.));
#5633=CARTESIAN_POINT('',(-2.1,0.7,0.6));
#5634=CARTESIAN_POINT('',(-2.1,0.,0.));
#5635=CARTESIAN_POINT('Origin',(2.1,0.,0.));
#5636=CARTESIAN_POINT('',(2.1,0.7,0.));
#5637=CARTESIAN_POINT('',(-2.1,0.7,0.));
#5638=CARTESIAN_POINT('',(2.1,0.,0.));
#5639=CARTESIAN_POINT('Origin',(2.1,0.,0.6));
#5640=CARTESIAN_POINT('',(2.1,0.7,0.));
#5641=CARTESIAN_POINT('Origin',(1.2,0.,3.75));
#5642=CARTESIAN_POINT('',(1.2,0.7,3.75));
#5643=CARTESIAN_POINT('',(1.2,0.7,0.6));
#5644=CARTESIAN_POINT('',(1.2,0.,3.75));
#5645=CARTESIAN_POINT('Origin',(0.1,0.,3.75));
#5646=CARTESIAN_POINT('',(0.1,0.7,3.75));
#5647=CARTESIAN_POINT('',(1.2,0.7,3.75));
#5648=CARTESIAN_POINT('',(0.1,0.,3.75));
#5649=CARTESIAN_POINT('Origin',(0.1,0.,2.95));
#5650=CARTESIAN_POINT('',(0.1,0.7,2.95));
#5651=CARTESIAN_POINT('',(0.1,0.7,3.75));
#5652=CARTESIAN_POINT('',(0.1,0.,2.95));
#5653=CARTESIAN_POINT('Origin',(-0.1,0.,2.95));
#5654=CARTESIAN_POINT('',(-0.1,0.7,2.95));
#5655=CARTESIAN_POINT('',(0.1,0.7,2.95));
#5656=CARTESIAN_POINT('',(-0.1,0.,2.95));
#5657=CARTESIAN_POINT('Origin',(-0.1,0.,3.75));
#5658=CARTESIAN_POINT('',(-0.1,0.7,3.75));
#5659=CARTESIAN_POINT('',(-0.1,0.7,2.95));
#5660=CARTESIAN_POINT('',(-0.1,0.,3.75));
#5661=CARTESIAN_POINT('Origin',(-1.2,0.,3.75));
#5662=CARTESIAN_POINT('',(-0.1,0.7,3.75));
#5663=CARTESIAN_POINT('Origin',(0.,0.7,1.875));
#6426=UNCERTAINTY_MEASURE_WITH_UNIT(LENGTH_MEASURE(0.001),#6464,
'DISTANCE_ACCURACY_VALUE',
'Maximum model space distance between geometric entities at asserted c
onnectivities');
#6442=UNCERTAINTY_MEASURE_WITH_UNIT(LENGTH_MEASURE(0.001),#6464,
'DISTANCE_ACCURACY_VALUE',
'Maximum model space distance between geometric entities at asserted c
onnectivities');
#6447=(
GEOMETRIC_REPRESENTATION_CONTEXT(3)
GLOBAL_UNCERTAINTY_ASSIGNED_CONTEXT((#6426))
GLOBAL_UNIT_ASSIGNED_CONTEXT((#6464,#6466,#6467))
REPRESENTATION_CONTEXT('','3D')
);
#6463=(
GEOMETRIC_REPRESENTATION_CONTEXT(3)
GLOBAL_UNCERTAINTY_ASSIGNED_CONTEXT((#6442))
GLOBAL_UNIT_ASSIGNED_CONTEXT((#6464,#6466,#6467))
REPRESENTATION_CONTEXT('','3D')
);
#6464=(
LENGTH_UNIT()
NAMED_UNIT(*)
SI_UNIT(.CENTI.,.METRE.)
);
#6466=(
NAMED_UNIT(*)
PLANE_ANGLE_UNIT()
SI_UNIT($,.RADIAN.)
);
#6467=(
NAMED_UNIT(*)
SI_UNIT($,.STERADIAN.)
SOLID_ANGLE_UNIT()
);
#6472=SHAPE_DEFINITION_REPRESENTATION(#6492,#6564);
#6492=PRODUCT_DEFINITION_SHAPE('',$,#6585);
#6564=SHAPE_REPRESENTATION('',(#3890),#6447);
#6580=PRODUCT_DEFINITION_CONTEXT('part definition',#6642,'design');
#6585=PRODUCT_DEFINITION('Relieved shaft support',
'Relieved shaft support',#6605,#6580);
#6605=PRODUCT_DEFINITION_FORMATION('',$,#6648);
#6642=APPLICATION_CONTEXT(
'Core Data for Automotive Mechanical Design Process');
#6643=PRODUCT_CONTEXT('part definition',#6642,'mechanical');
#6648=PRODUCT('Relieved shaft support','Relieved shaft support',
'Relieved shaft support',(#6643));
#6734=COLOUR_RGB('Grey',0.48,0.52,0.57);
#6735=FILL_AREA_STYLE_COLOUR('',#6734);
#6736=FILL_AREA_STYLE('',(#6735));
#6737=SURFACE_STYLE_FILL_AREA(#6736);
#6738=SURFACE_SIDE_STYLE('',(#6737));
#6739=SURFACE_STYLE_USAGE(.BOTH.,#6738);
#6740=PRESENTATION_STYLE_ASSIGNMENT((#6739));
ENDSEC;
END-ISO-10303-21;
